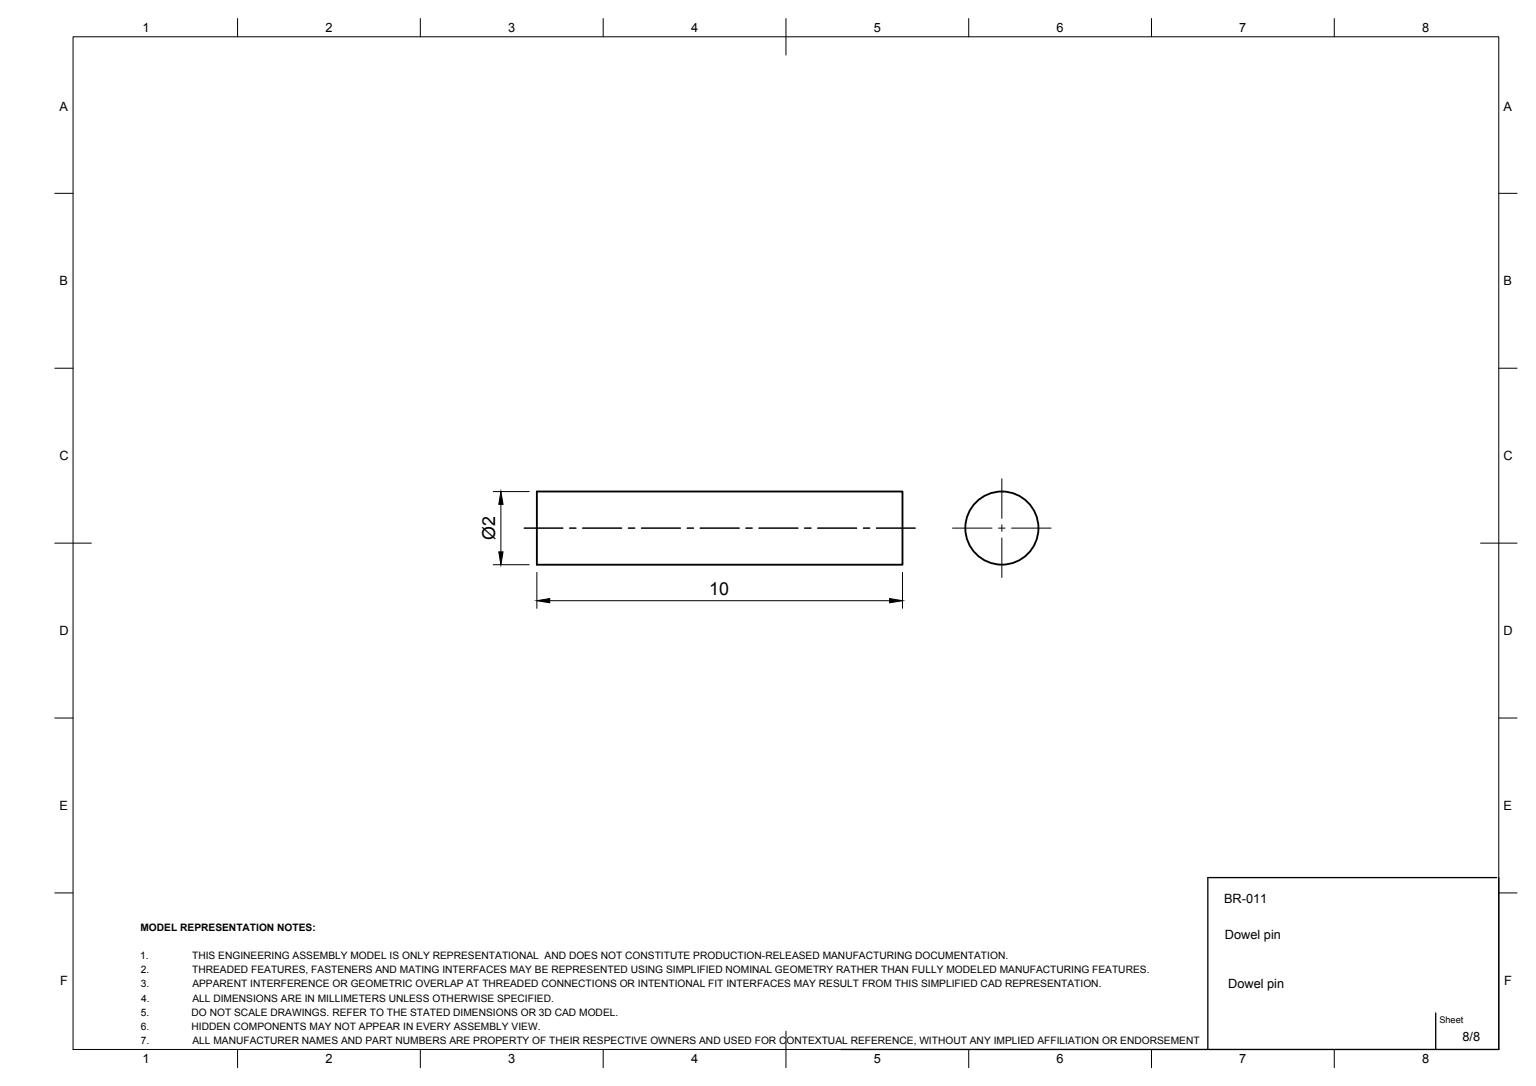
ISO-10303-21;
HEADER;
/* Generated by software containing ST-Developer
 * from STEP Tools, Inc. (www.steptools.com) 
 */

FILE_DESCRIPTION(
/* description */ ('Independent pair of monolithic parallel-leaf compliant finger modules.
 Shared native part/module instances; external gripper actuator outsid
e scope. Whole-mm geometry,1mm webs,56mm straight span,12mm depth,32mm
 nominal contact gap. Undeformed CAD reference; material condition, el
astic range, fatigue and gripping force unassigned.'),
/* implementation_level */ '2;1');

FILE_NAME(
/* name */ 'Dowel pin.step',
/* time_stamp */ '2026-11-07T22:36:16-08:00',
/* author */ (''),
/* organization */ (''),
/* preprocessor_version */ 'ST-DEVELOPER v20.2',
/* originating_system */ 'Autodesk Translation Framework v15.17.0.0',
/* authorisation */ '');

FILE_SCHEMA (('AUTOMOTIVE_DESIGN { 1 0 10303 214 3 1 1 }'));
ENDSEC;

DATA;
#10=MECHANICAL_DESIGN_GEOMETRIC_PRESENTATION_REPRESENTATION('',(#334),#13801);
#322=SHAPE_REPRESENTATION_RELATIONSHIP('SRR','None',#13840,#328);
#328=ADVANCED_BREP_SHAPE_REPRESENTATION('',(#340),#13800);
#334=STYLED_ITEM('',(#13883),#340);
#340=MANIFOLD_SOLID_BREP('Body1',#3699);
#415=PLANE('',#4027);
#416=PLANE('',#4028);
#615=FACE_OUTER_BOUND('',#840,.T.);
#616=FACE_OUTER_BOUND('',#841,.T.);
#617=FACE_OUTER_BOUND('',#842,.T.);
#840=EDGE_LOOP('',(#3345,#3346,#3347,#3348));
#841=EDGE_LOOP('',(#3349));
#842=EDGE_LOOP('',(#3350));
#1071=LINE('',#13769,#1300);
#1300=VECTOR('',#4786,1.);
#1358=CIRCLE('',#4025,1.);
#1359=CIRCLE('',#4026,1.);
#1720=VERTEX_POINT('',#13766);
#1721=VERTEX_POINT('',#13768);
#2262=EDGE_CURVE('',#1720,#1720,#1358,.T.);
#2263=EDGE_CURVE('',#1720,#1721,#1071,.T.);
#2264=EDGE_CURVE('',#1721,#1721,#1359,.T.);
#3345=ORIENTED_EDGE('',*,*,#2262,.F.);
#3346=ORIENTED_EDGE('',*,*,#2263,.T.);
#3347=ORIENTED_EDGE('',*,*,#2264,.T.);
#3348=ORIENTED_EDGE('',*,*,#2263,.F.);
#3349=ORIENTED_EDGE('',*,*,#2262,.T.);
#3350=ORIENTED_EDGE('',*,*,#2264,.F.);
#3492=CYLINDRICAL_SURFACE('',#4024,1.);
#3691=ADVANCED_FACE('',(#615),#3492,.T.);
#3692=ADVANCED_FACE('',(#616),#415,.T.);
#3693=ADVANCED_FACE('',(#617),#416,.F.);
#3699=CLOSED_SHELL('',(#3691,#3692,#3693));
#4023=AXIS2_PLACEMENT_3D('',#13764,#4780,#4781);
#4024=AXIS2_PLACEMENT_3D('',#13765,#4782,#4783);
#4025=AXIS2_PLACEMENT_3D('',#13767,#4784,#4785);
#4026=AXIS2_PLACEMENT_3D('',#13770,#4787,#4788);
#4027=AXIS2_PLACEMENT_3D('',#13771,#4789,#4790);
#4028=AXIS2_PLACEMENT_3D('',#13772,#4791,#4792);
#4780=DIRECTION('axis',(0.,0.,1.));
#4781=DIRECTION('refdir',(1.,0.,0.));
#4782=DIRECTION('center_axis',(0.,0.,1.));
#4783=DIRECTION('ref_axis',(1.,0.,0.));
#4784=DIRECTION('center_axis',(0.,0.,1.));
#4785=DIRECTION('ref_axis',(1.,0.,0.));
#4786=DIRECTION('',(0.,0.,-1.));
#4787=DIRECTION('center_axis',(0.,0.,1.));
#4788=DIRECTION('ref_axis',(1.,0.,0.));
#4789=DIRECTION('center_axis',(0.,0.,1.));
#4790=DIRECTION('ref_axis',(1.,0.,0.));
#4791=DIRECTION('center_axis',(0.,0.,1.));
#4792=DIRECTION('ref_axis',(1.,0.,0.));
#13764=CARTESIAN_POINT('',(0.,0.,0.));
#13765=CARTESIAN_POINT('Origin',(0.,0.,0.));
#13766=CARTESIAN_POINT('',(-1.,-1.22464679914735E-16,10.));
#13767=CARTESIAN_POINT('Origin',(0.,0.,10.));
#13768=CARTESIAN_POINT('',(-1.,-1.22464679914735E-16,0.));
#13769=CARTESIAN_POINT('',(-1.,-1.22464679914735E-16,0.));
#13770=CARTESIAN_POINT('Origin',(0.,0.,0.));
#13771=CARTESIAN_POINT('Origin',(0.,0.,10.));
#13772=CARTESIAN_POINT('Origin',(0.,0.,0.));
#13791=UNCERTAINTY_MEASURE_WITH_UNIT(LENGTH_MEASURE(0.01),#13802,
'DISTANCE_ACCURACY_VALUE',
'Maximum model space distance between geometric entities at asserted c
onnectivities');
#13792=UNCERTAINTY_MEASURE_WITH_UNIT(LENGTH_MEASURE(0.01),#13802,
'DISTANCE_ACCURACY_VALUE',
'Maximum model space distance between geometric entities at asserted c
onnectivities');
#13800=(
GEOMETRIC_REPRESENTATION_CONTEXT(3)
GLOBAL_UNCERTAINTY_ASSIGNED_CONTEXT((#13791))
GLOBAL_UNIT_ASSIGNED_CONTEXT((#13802,#13804,#13805))
REPRESENTATION_CONTEXT('','3D')
);
#13801=(
GEOMETRIC_REPRESENTATION_CONTEXT(3)
GLOBAL_UNCERTAINTY_ASSIGNED_CONTEXT((#13792))
GLOBAL_UNIT_ASSIGNED_CONTEXT((#13802,#13804,#13805))
REPRESENTATION_CONTEXT('','3D')
);
#13802=(
LENGTH_UNIT()
NAMED_UNIT(*)
SI_UNIT(.MILLI.,.METRE.)
);
#13804=(
NAMED_UNIT(*)
PLANE_ANGLE_UNIT()
SI_UNIT($,.RADIAN.)
);
#13805=(
NAMED_UNIT(*)
SI_UNIT($,.STERADIAN.)
SOLID_ANGLE_UNIT()
);
#13813=SHAPE_DEFINITION_REPRESENTATION(#13821,#13840);
#13821=PRODUCT_DEFINITION_SHAPE('',$,#13849);
#13840=SHAPE_REPRESENTATION('',(#4023),#13800);
#13841=PRODUCT_DEFINITION_CONTEXT('part definition',#13867,'design');
#13849=PRODUCT_DEFINITION('Dowel pin','Dowel pin',#13857,#13841);
#13857=PRODUCT_DEFINITION_FORMATION('',$,#13876);
#13867=APPLICATION_CONTEXT(
'Core Data for Automotive Mechanical Design Process');
#13868=PRODUCT_CONTEXT('part definition',#13867,'mechanical');
#13876=PRODUCT('Dowel pin','Dowel pin',$,(#13868));
#13883=PRESENTATION_STYLE_ASSIGNMENT((#13890));
#13890=SURFACE_STYLE_USAGE(.BOTH.,#13897);
#13897=SURFACE_SIDE_STYLE('',(#13904));
#13904=SURFACE_STYLE_FILL_AREA(#13911);
#13911=FILL_AREA_STYLE('Gray',(#13918));
#13918=FILL_AREA_STYLE_COLOUR('Gray',#13925);
#13925=COLOUR_RGB('Gray',0.407843137254902,0.447058823529412,0.498039215686275);
ENDSEC;
END-ISO-10303-21;
